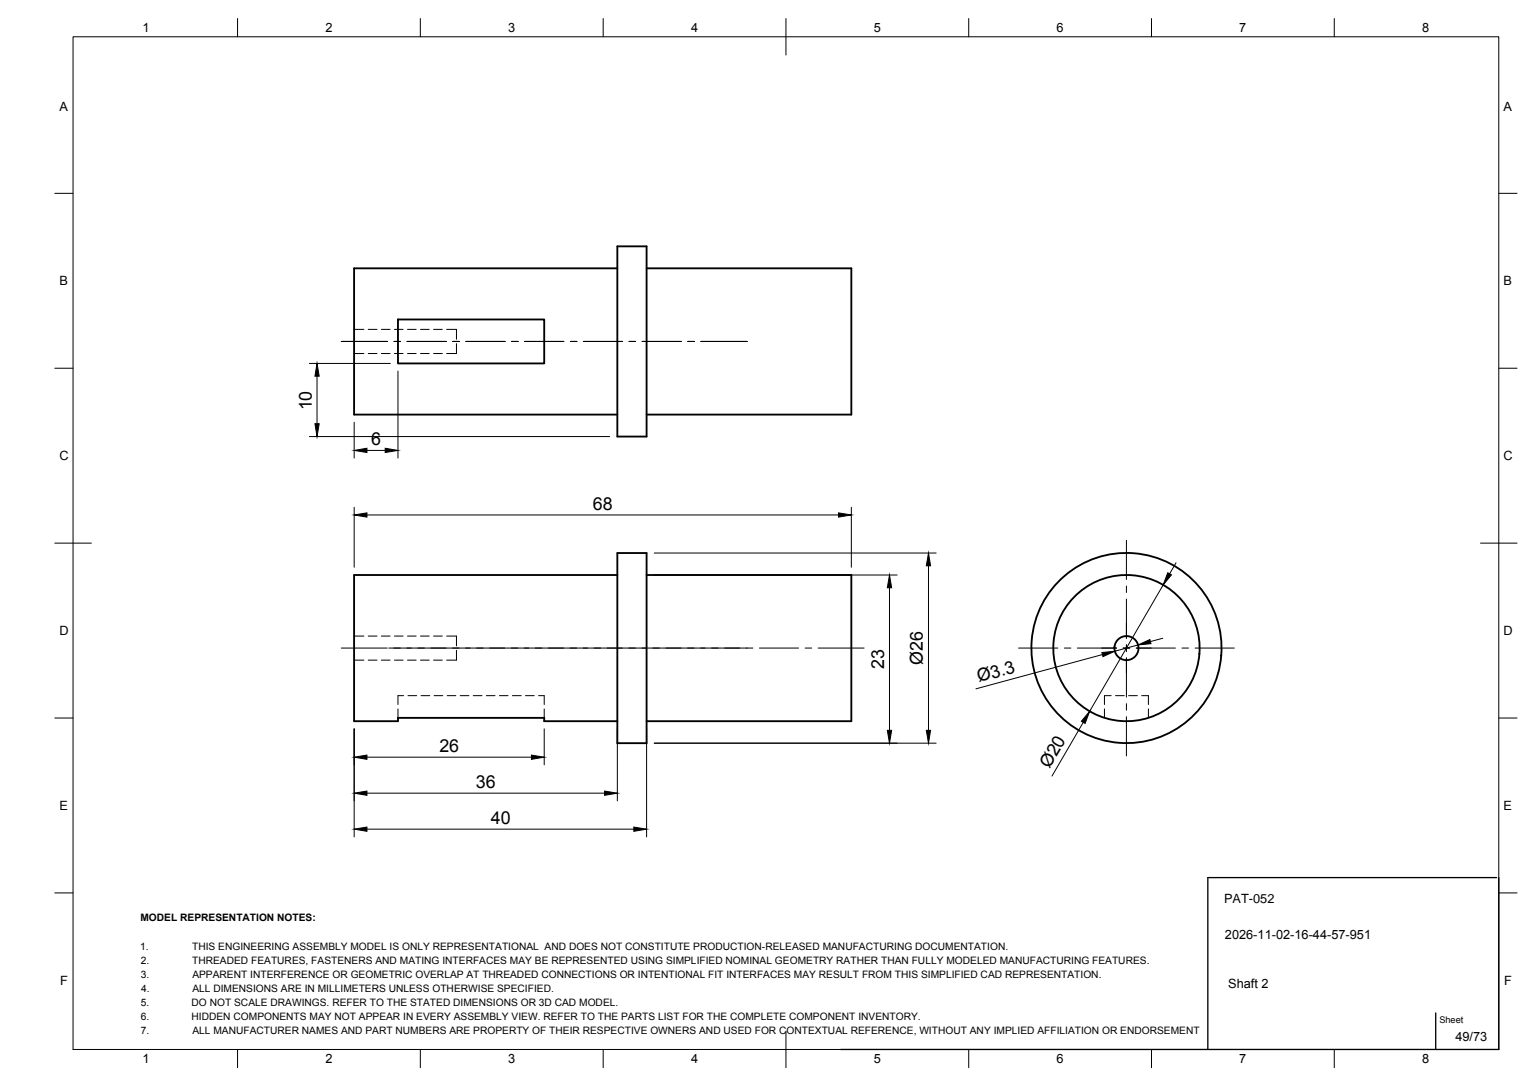
ISO-10303-21;
HEADER;
/* Generated by software containing ST-Developer
 * from STEP Tools, Inc. (www.steptools.com) 
 */

FILE_DESCRIPTION(
/* description */ ('Hand-crank gear train demonstrator'),
/* implementation_level */ '2;1');

FILE_NAME(
/* name */ 'Shaft 2.step',
/* time_stamp */ '2026-10-28T03:22:13-07:00',
/* author */ (''),
/* organization */ (''),
/* preprocessor_version */ 'ST-DEVELOPER v20.2',
/* originating_system */ 'Autodesk Translation Framework v15.17.0.0',
/* authorisation */ '');

FILE_SCHEMA (('AUTOMOTIVE_DESIGN { 1 0 10303 214 3 1 1 }'));
ENDSEC;

DATA;
#10=MECHANICAL_DESIGN_GEOMETRIC_PRESENTATION_REPRESENTATION('',(#1243),#62758);
#1100=SHAPE_REPRESENTATION_RELATIONSHIP('SRR','None',#63076,#1164);
#1164=ADVANCED_BREP_SHAPE_REPRESENTATION('',(#1318),#62730);
#1243=STYLED_ITEM('',(#63462),#1318);
#1318=MANIFOLD_SOLID_BREP('Body1',#16427);
#1572=FACE_BOUND('',#3806,.T.);
#1573=FACE_BOUND('',#3808,.T.);
#1574=FACE_BOUND('',#3812,.T.);
#1575=FACE_BOUND('',#3814,.T.);
#1937=PLANE('',#18140);
#1938=PLANE('',#18141);
#1939=PLANE('',#18142);
#1940=PLANE('',#18144);
#1941=PLANE('',#18145);
#1942=PLANE('',#18146);
#1943=PLANE('',#18148);
#1944=PLANE('',#18151);
#1945=PLANE('',#18159);
#1946=PLANE('',#18160);
#2632=FACE_OUTER_BOUND('',#3798,.T.);
#2633=FACE_OUTER_BOUND('',#3799,.T.);
#2634=FACE_OUTER_BOUND('',#3800,.T.);
#2635=FACE_OUTER_BOUND('',#3801,.T.);
#2636=FACE_OUTER_BOUND('',#3802,.T.);
#2637=FACE_OUTER_BOUND('',#3803,.T.);
#2638=FACE_OUTER_BOUND('',#3804,.T.);
#2639=FACE_OUTER_BOUND('',#3805,.T.);
#2640=FACE_OUTER_BOUND('',#3807,.T.);
#2641=FACE_OUTER_BOUND('',#3809,.T.);
#2642=FACE_OUTER_BOUND('',#3810,.T.);
#2643=FACE_OUTER_BOUND('',#3811,.T.);
#2644=FACE_OUTER_BOUND('',#3813,.T.);
#2645=FACE_OUTER_BOUND('',#3815,.T.);
#3798=EDGE_LOOP('',(#13023,#13024,#13025,#13026));
#3799=EDGE_LOOP('',(#13027));
#3800=EDGE_LOOP('',(#13028,#13029,#13030,#13031));
#3801=EDGE_LOOP('',(#13032,#13033,#13034,#13035));
#3802=EDGE_LOOP('',(#13036,#13037,#13038,#13039));
#3803=EDGE_LOOP('',(#13040,#13041,#13042,#13043));
#3804=EDGE_LOOP('',(#13044,#13045,#13046,#13047));
#3805=EDGE_LOOP('',(#13048));
#3806=EDGE_LOOP('',(#13049));
#3807=EDGE_LOOP('',(#13050));
#3808=EDGE_LOOP('',(#13051));
#3809=EDGE_LOOP('',(#13052,#13053,#13054,#13055));
#3810=EDGE_LOOP('',(#13056,#13057,#13058,#13059));
#3811=EDGE_LOOP('',(#13060,#13061,#13062,#13063));
#3812=EDGE_LOOP('',(#13064,#13065,#13066,#13067));
#3813=EDGE_LOOP('',(#13068));
#3814=EDGE_LOOP('',(#13069));
#3815=EDGE_LOOP('',(#13070));
#4930=LINE('',#26399,#6062);
#4931=LINE('',#26405,#6063);
#4932=LINE('',#26407,#6064);
#4933=LINE('',#26409,#6065);
#4934=LINE('',#26410,#6066);
#4935=LINE('',#26415,#6067);
#4936=LINE('',#26416,#6068);
#4937=LINE('',#26419,#6069);
#4938=LINE('',#26421,#6070);
#4939=LINE('',#26422,#6071);
#4940=LINE('',#26424,#6072);
#4941=LINE('',#26438,#6073);
#4942=LINE('',#26441,#6074);
#4943=LINE('',#26446,#6075);
#6062=VECTOR('',#21437,0.165);
#6063=VECTOR('',#21444,1.);
#6064=VECTOR('',#21445,1.);
#6065=VECTOR('',#21446,1.);
#6066=VECTOR('',#21447,1.);
#6067=VECTOR('',#21452,1.);
#6068=VECTOR('',#21453,1.);
#6069=VECTOR('',#21456,1.);
#6070=VECTOR('',#21457,1.);
#6071=VECTOR('',#21458,1.);
#6072=VECTOR('',#21461,1.);
#6073=VECTOR('',#21480,1.3);
#6074=VECTOR('',#21483,1.);
#6075=VECTOR('',#21490,1.);
#6964=CIRCLE('',#18138,0.165);
#6965=CIRCLE('',#18139,0.165);
#6966=CIRCLE('',#18143,1.);
#6967=CIRCLE('',#18147,1.);
#6968=CIRCLE('',#18149,1.3);
#6969=CIRCLE('',#18150,1.);
#6970=CIRCLE('',#18152,1.3);
#6971=CIRCLE('',#18153,1.);
#6972=CIRCLE('',#18156,1.);
#6973=CIRCLE('',#18158,1.);
#7955=VERTEX_POINT('',#26396);
#7956=VERTEX_POINT('',#26398);
#7957=VERTEX_POINT('',#26403);
#7958=VERTEX_POINT('',#26404);
#7959=VERTEX_POINT('',#26406);
#7960=VERTEX_POINT('',#26408);
#7961=VERTEX_POINT('',#26412);
#7962=VERTEX_POINT('',#26414);
#7963=VERTEX_POINT('',#26418);
#7964=VERTEX_POINT('',#26420);
#7965=VERTEX_POINT('',#26428);
#7966=VERTEX_POINT('',#26430);
#7967=VERTEX_POINT('',#26433);
#7968=VERTEX_POINT('',#26435);
#7969=VERTEX_POINT('',#26440);
#7970=VERTEX_POINT('',#26444);
#9763=EDGE_CURVE('',#7955,#7955,#6964,.T.);
#9764=EDGE_CURVE('',#7955,#7956,#4930,.T.);
#9765=EDGE_CURVE('',#7956,#7956,#6965,.T.);
#9766=EDGE_CURVE('',#7957,#7958,#4931,.T.);
#9767=EDGE_CURVE('',#7957,#7959,#4932,.T.);
#9768=EDGE_CURVE('',#7960,#7959,#4933,.T.);
#9769=EDGE_CURVE('',#7960,#7958,#4934,.T.);
#9770=EDGE_CURVE('',#7958,#7961,#6966,.T.);
#9771=EDGE_CURVE('',#7962,#7960,#4935,.T.);
#9772=EDGE_CURVE('',#7961,#7962,#4936,.T.);
#9773=EDGE_CURVE('',#7961,#7963,#4937,.T.);
#9774=EDGE_CURVE('',#7962,#7964,#4938,.T.);
#9775=EDGE_CURVE('',#7964,#7963,#4939,.T.);
#9776=EDGE_CURVE('',#7959,#7964,#4940,.T.);
#9777=EDGE_CURVE('',#7963,#7957,#6967,.T.);
#9778=EDGE_CURVE('',#7965,#7965,#6968,.T.);
#9779=EDGE_CURVE('',#7966,#7966,#6969,.T.);
#9780=EDGE_CURVE('',#7967,#7967,#6970,.T.);
#9781=EDGE_CURVE('',#7968,#7968,#6971,.T.);
#9782=EDGE_CURVE('',#7965,#7967,#4941,.T.);
#9783=EDGE_CURVE('',#7968,#7969,#4942,.T.);
#9784=EDGE_CURVE('',#7969,#7969,#6972,.T.);
#9785=EDGE_CURVE('',#7970,#7970,#6973,.T.);
#9786=EDGE_CURVE('',#7970,#7966,#4943,.T.);
#13023=ORIENTED_EDGE('',*,*,#9763,.F.);
#13024=ORIENTED_EDGE('',*,*,#9764,.T.);
#13025=ORIENTED_EDGE('',*,*,#9765,.F.);
#13026=ORIENTED_EDGE('',*,*,#9764,.F.);
#13027=ORIENTED_EDGE('',*,*,#9763,.T.);
#13028=ORIENTED_EDGE('',*,*,#9766,.F.);
#13029=ORIENTED_EDGE('',*,*,#9767,.T.);
#13030=ORIENTED_EDGE('',*,*,#9768,.F.);
#13031=ORIENTED_EDGE('',*,*,#9769,.T.);
#13032=ORIENTED_EDGE('',*,*,#9770,.F.);
#13033=ORIENTED_EDGE('',*,*,#9769,.F.);
#13034=ORIENTED_EDGE('',*,*,#9771,.F.);
#13035=ORIENTED_EDGE('',*,*,#9772,.F.);
#13036=ORIENTED_EDGE('',*,*,#9773,.F.);
#13037=ORIENTED_EDGE('',*,*,#9772,.T.);
#13038=ORIENTED_EDGE('',*,*,#9774,.T.);
#13039=ORIENTED_EDGE('',*,*,#9775,.T.);
#13040=ORIENTED_EDGE('',*,*,#9771,.T.);
#13041=ORIENTED_EDGE('',*,*,#9768,.T.);
#13042=ORIENTED_EDGE('',*,*,#9776,.T.);
#13043=ORIENTED_EDGE('',*,*,#9774,.F.);
#13044=ORIENTED_EDGE('',*,*,#9777,.F.);
#13045=ORIENTED_EDGE('',*,*,#9775,.F.);
#13046=ORIENTED_EDGE('',*,*,#9776,.F.);
#13047=ORIENTED_EDGE('',*,*,#9767,.F.);
#13048=ORIENTED_EDGE('',*,*,#9778,.T.);
#13049=ORIENTED_EDGE('',*,*,#9779,.F.);
#13050=ORIENTED_EDGE('',*,*,#9780,.F.);
#13051=ORIENTED_EDGE('',*,*,#9781,.F.);
#13052=ORIENTED_EDGE('',*,*,#9778,.F.);
#13053=ORIENTED_EDGE('',*,*,#9782,.T.);
#13054=ORIENTED_EDGE('',*,*,#9780,.T.);
#13055=ORIENTED_EDGE('',*,*,#9782,.F.);
#13056=ORIENTED_EDGE('',*,*,#9781,.T.);
#13057=ORIENTED_EDGE('',*,*,#9783,.T.);
#13058=ORIENTED_EDGE('',*,*,#9784,.T.);
#13059=ORIENTED_EDGE('',*,*,#9783,.F.);
#13060=ORIENTED_EDGE('',*,*,#9785,.F.);
#13061=ORIENTED_EDGE('',*,*,#9786,.T.);
#13062=ORIENTED_EDGE('',*,*,#9779,.T.);
#13063=ORIENTED_EDGE('',*,*,#9786,.F.);
#13064=ORIENTED_EDGE('',*,*,#9773,.T.);
#13065=ORIENTED_EDGE('',*,*,#9777,.T.);
#13066=ORIENTED_EDGE('',*,*,#9766,.T.);
#13067=ORIENTED_EDGE('',*,*,#9770,.T.);
#13068=ORIENTED_EDGE('',*,*,#9785,.T.);
#13069=ORIENTED_EDGE('',*,*,#9765,.T.);
#13070=ORIENTED_EDGE('',*,*,#9784,.F.);
#15318=CYLINDRICAL_SURFACE('',#18137,0.165);
#15319=CYLINDRICAL_SURFACE('',#18154,1.3);
#15320=CYLINDRICAL_SURFACE('',#18155,1.);
#15321=CYLINDRICAL_SURFACE('',#18157,1.);
#15942=ADVANCED_FACE('',(#2632),#15318,.F.);
#15943=ADVANCED_FACE('',(#2633),#1937,.T.);
#15944=ADVANCED_FACE('',(#2634),#1938,.F.);
#15945=ADVANCED_FACE('',(#2635),#1939,.T.);
#15946=ADVANCED_FACE('',(#2636),#1940,.F.);
#15947=ADVANCED_FACE('',(#2637),#1941,.F.);
#15948=ADVANCED_FACE('',(#2638),#1942,.F.);
#15949=ADVANCED_FACE('',(#2639,#1572),#1943,.T.);
#15950=ADVANCED_FACE('',(#2640,#1573),#1944,.F.);
#15951=ADVANCED_FACE('',(#2641),#15319,.T.);
#15952=ADVANCED_FACE('',(#2642),#15320,.T.);
#15953=ADVANCED_FACE('',(#2643,#1574),#15321,.T.);
#15954=ADVANCED_FACE('',(#2644,#1575),#1945,.T.);
#15955=ADVANCED_FACE('',(#2645),#1946,.F.);
#16427=CLOSED_SHELL('',(#15942,#15943,#15944,#15945,#15946,#15947,#15948,
#15949,#15950,#15951,#15952,#15953,#15954,#15955));
#18136=AXIS2_PLACEMENT_3D('',#26394,#21431,#21432);
#18137=AXIS2_PLACEMENT_3D('',#26395,#21433,#21434);
#18138=AXIS2_PLACEMENT_3D('',#26397,#21435,#21436);
#18139=AXIS2_PLACEMENT_3D('',#26400,#21438,#21439);
#18140=AXIS2_PLACEMENT_3D('',#26401,#21440,#21441);
#18141=AXIS2_PLACEMENT_3D('',#26402,#21442,#21443);
#18142=AXIS2_PLACEMENT_3D('',#26411,#21448,#21449);
#18143=AXIS2_PLACEMENT_3D('',#26413,#21450,#21451);
#18144=AXIS2_PLACEMENT_3D('',#26417,#21454,#21455);
#18145=AXIS2_PLACEMENT_3D('',#26423,#21459,#21460);
#18146=AXIS2_PLACEMENT_3D('',#26425,#21462,#21463);
#18147=AXIS2_PLACEMENT_3D('',#26426,#21464,#21465);
#18148=AXIS2_PLACEMENT_3D('',#26427,#21466,#21467);
#18149=AXIS2_PLACEMENT_3D('',#26429,#21468,#21469);
#18150=AXIS2_PLACEMENT_3D('',#26431,#21470,#21471);
#18151=AXIS2_PLACEMENT_3D('',#26432,#21472,#21473);
#18152=AXIS2_PLACEMENT_3D('',#26434,#21474,#21475);
#18153=AXIS2_PLACEMENT_3D('',#26436,#21476,#21477);
#18154=AXIS2_PLACEMENT_3D('',#26437,#21478,#21479);
#18155=AXIS2_PLACEMENT_3D('',#26439,#21481,#21482);
#18156=AXIS2_PLACEMENT_3D('',#26442,#21484,#21485);
#18157=AXIS2_PLACEMENT_3D('',#26443,#21486,#21487);
#18158=AXIS2_PLACEMENT_3D('',#26445,#21488,#21489);
#18159=AXIS2_PLACEMENT_3D('',#26447,#21491,#21492);
#18160=AXIS2_PLACEMENT_3D('',#26448,#21493,#21494);
#21431=DIRECTION('axis',(0.,0.,1.));
#21432=DIRECTION('refdir',(1.,0.,0.));
#21433=DIRECTION('center_axis',(0.,1.,0.));
#21434=DIRECTION('ref_axis',(1.,0.,0.));
#21435=DIRECTION('center_axis',(0.,1.,0.));
#21436=DIRECTION('ref_axis',(1.,0.,0.));
#21437=DIRECTION('',(0.,1.,0.));
#21438=DIRECTION('center_axis',(0.,-1.,0.));
#21439=DIRECTION('ref_axis',(1.,0.,0.));
#21440=DIRECTION('center_axis',(0.,1.,0.));
#21441=DIRECTION('ref_axis',(1.,0.,0.));
#21442=DIRECTION('center_axis',(-1.,0.,0.));
#21443=DIRECTION('ref_axis',(0.,0.,1.));
#21444=DIRECTION('',(0.,-1.,0.));
#21445=DIRECTION('',(0.,0.,1.));
#21446=DIRECTION('',(0.,1.,0.));
#21447=DIRECTION('',(0.,0.,-1.));
#21448=DIRECTION('center_axis',(0.,1.,0.));
#21449=DIRECTION('ref_axis',(1.,0.,0.));
#21450=DIRECTION('center_axis',(0.,-1.,0.));
#21451=DIRECTION('ref_axis',(1.,0.,0.));
#21452=DIRECTION('',(-1.,0.,0.));
#21453=DIRECTION('',(0.,0.,1.));
#21454=DIRECTION('center_axis',(1.,0.,0.));
#21455=DIRECTION('ref_axis',(0.,0.,-1.));
#21456=DIRECTION('',(0.,1.,0.));
#21457=DIRECTION('',(0.,1.,0.));
#21458=DIRECTION('',(0.,0.,-1.));
#21459=DIRECTION('center_axis',(0.,0.,1.));
#21460=DIRECTION('ref_axis',(1.,0.,0.));
#21461=DIRECTION('',(1.,0.,0.));
#21462=DIRECTION('center_axis',(0.,1.,0.));
#21463=DIRECTION('ref_axis',(0.,0.,1.));
#21464=DIRECTION('center_axis',(0.,1.,0.));
#21465=DIRECTION('ref_axis',(1.,0.,0.));
#21466=DIRECTION('center_axis',(0.,1.,0.));
#21467=DIRECTION('ref_axis',(1.,0.,0.));
#21468=DIRECTION('center_axis',(0.,1.,0.));
#21469=DIRECTION('ref_axis',(1.,0.,0.));
#21470=DIRECTION('center_axis',(0.,1.,0.));
#21471=DIRECTION('ref_axis',(1.,0.,0.));
#21472=DIRECTION('center_axis',(0.,1.,0.));
#21473=DIRECTION('ref_axis',(1.,0.,0.));
#21474=DIRECTION('center_axis',(0.,1.,0.));
#21475=DIRECTION('ref_axis',(1.,0.,0.));
#21476=DIRECTION('center_axis',(0.,-1.,0.));
#21477=DIRECTION('ref_axis',(1.,0.,0.));
#21478=DIRECTION('center_axis',(0.,1.,0.));
#21479=DIRECTION('ref_axis',(1.,0.,0.));
#21480=DIRECTION('',(0.,-1.,0.));
#21481=DIRECTION('center_axis',(0.,1.,0.));
#21482=DIRECTION('ref_axis',(1.,0.,0.));
#21483=DIRECTION('',(0.,-1.,0.));
#21484=DIRECTION('center_axis',(0.,1.,0.));
#21485=DIRECTION('ref_axis',(1.,0.,0.));
#21486=DIRECTION('center_axis',(0.,1.,0.));
#21487=DIRECTION('ref_axis',(1.,0.,0.));
#21488=DIRECTION('center_axis',(0.,1.,0.));
#21489=DIRECTION('ref_axis',(1.,0.,0.));
#21490=DIRECTION('',(0.,-1.,0.));
#21491=DIRECTION('center_axis',(0.,1.,0.));
#21492=DIRECTION('ref_axis',(1.,0.,0.));
#21493=DIRECTION('center_axis',(0.,1.,0.));
#21494=DIRECTION('ref_axis',(1.,0.,0.));
#26394=CARTESIAN_POINT('',(0.,0.,0.));
#26395=CARTESIAN_POINT('Origin',(6.,1.8,9.));
#26396=CARTESIAN_POINT('',(5.835,1.8,9.));
#26397=CARTESIAN_POINT('Origin',(6.,1.8,9.));
#26398=CARTESIAN_POINT('',(5.835,3.2,9.));
#26399=CARTESIAN_POINT('',(5.835,1.8,9.));
#26400=CARTESIAN_POINT('Origin',(6.,3.2,9.));
#26401=CARTESIAN_POINT('Origin',(6.,1.8,9.));
#26402=CARTESIAN_POINT('Origin',(5.7,0.6,7.));
#26403=CARTESIAN_POINT('',(5.7,2.6,8.04606079858305));
#26404=CARTESIAN_POINT('',(5.7,0.6,8.04606079858305));
#26405=CARTESIAN_POINT('',(5.7,-3.6,8.04606079858305));
#26406=CARTESIAN_POINT('',(5.7,2.6,8.35));
#26407=CARTESIAN_POINT('',(5.7,2.6,8.35));
#26408=CARTESIAN_POINT('',(5.7,0.6,8.35));
#26409=CARTESIAN_POINT('',(5.7,0.6,8.35));
#26410=CARTESIAN_POINT('',(5.7,0.6,8.35));
#26411=CARTESIAN_POINT('Origin',(6.,0.6,7.675));
#26412=CARTESIAN_POINT('',(6.3,0.6,8.04606079858305));
#26413=CARTESIAN_POINT('Origin',(6.,0.6,9.));
#26414=CARTESIAN_POINT('',(6.3,0.6,8.35));
#26415=CARTESIAN_POINT('',(6.3,0.6,8.35));
#26416=CARTESIAN_POINT('',(6.3,0.6,7.));
#26417=CARTESIAN_POINT('Origin',(6.3,0.6,8.35));
#26418=CARTESIAN_POINT('',(6.3,2.6,8.04606079858305));
#26419=CARTESIAN_POINT('',(6.3,-3.6,8.04606079858305));
#26420=CARTESIAN_POINT('',(6.3,2.6,8.35));
#26421=CARTESIAN_POINT('',(6.3,0.6,8.35));
#26422=CARTESIAN_POINT('',(6.3,2.6,7.));
#26423=CARTESIAN_POINT('Origin',(5.7,0.6,8.35));
#26424=CARTESIAN_POINT('',(6.3,2.6,8.35));
#26425=CARTESIAN_POINT('Origin',(6.,2.6,7.675));
#26426=CARTESIAN_POINT('Origin',(6.,2.6,9.));
#26427=CARTESIAN_POINT('Origin',(6.,-0.4,9.));
#26428=CARTESIAN_POINT('',(4.7,-0.4,9.));
#26429=CARTESIAN_POINT('Origin',(6.,-0.4,9.));
#26430=CARTESIAN_POINT('',(5.,-0.4,9.));
#26431=CARTESIAN_POINT('Origin',(6.,-0.4,9.));
#26432=CARTESIAN_POINT('Origin',(6.,-0.8,9.));
#26433=CARTESIAN_POINT('',(4.7,-0.8,9.));
#26434=CARTESIAN_POINT('Origin',(6.,-0.8,9.));
#26435=CARTESIAN_POINT('',(5.,-0.8,9.));
#26436=CARTESIAN_POINT('Origin',(6.,-0.8,9.));
#26437=CARTESIAN_POINT('Origin',(6.,-0.8,9.));
#26438=CARTESIAN_POINT('',(4.7,-0.8,9.));
#26439=CARTESIAN_POINT('Origin',(6.,-3.6,9.));
#26440=CARTESIAN_POINT('',(5.,-3.6,9.));
#26441=CARTESIAN_POINT('',(5.,-3.6,9.));
#26442=CARTESIAN_POINT('Origin',(6.,-3.6,9.));
#26443=CARTESIAN_POINT('Origin',(6.,-3.6,9.));
#26444=CARTESIAN_POINT('',(5.,3.2,9.));
#26445=CARTESIAN_POINT('Origin',(6.,3.2,9.));
#26446=CARTESIAN_POINT('',(5.,-3.6,9.));
#26447=CARTESIAN_POINT('Origin',(6.,3.2,9.));
#26448=CARTESIAN_POINT('Origin',(6.,-3.6,9.));
#62656=UNCERTAINTY_MEASURE_WITH_UNIT(LENGTH_MEASURE(0.001),#62759,
'DISTANCE_ACCURACY_VALUE',
'Maximum model space distance between geometric entities at asserted c
onnectivities');
#62684=UNCERTAINTY_MEASURE_WITH_UNIT(LENGTH_MEASURE(0.001),#62759,
'DISTANCE_ACCURACY_VALUE',
'Maximum model space distance between geometric entities at asserted c
onnectivities');
#62730=(
GEOMETRIC_REPRESENTATION_CONTEXT(3)
GLOBAL_UNCERTAINTY_ASSIGNED_CONTEXT((#62656))
GLOBAL_UNIT_ASSIGNED_CONTEXT((#62759,#62761,#62762))
REPRESENTATION_CONTEXT('','3D')
);
#62758=(
GEOMETRIC_REPRESENTATION_CONTEXT(3)
GLOBAL_UNCERTAINTY_ASSIGNED_CONTEXT((#62684))
GLOBAL_UNIT_ASSIGNED_CONTEXT((#62759,#62761,#62762))
REPRESENTATION_CONTEXT('','3D')
);
#62759=(
LENGTH_UNIT()
NAMED_UNIT(*)
SI_UNIT(.CENTI.,.METRE.)
);
#62761=(
NAMED_UNIT(*)
PLANE_ANGLE_UNIT()
SI_UNIT($,.RADIAN.)
);
#62762=(
NAMED_UNIT(*)
SI_UNIT($,.STERADIAN.)
SOLID_ANGLE_UNIT()
);
#62808=SHAPE_DEFINITION_REPRESENTATION(#62891,#63076);
#62891=PRODUCT_DEFINITION_SHAPE('',$,#63150);
#63076=SHAPE_REPRESENTATION('',(#18136),#62730);
#63104=PRODUCT_DEFINITION_CONTEXT('part definition',#63325,'design');
#63150=PRODUCT_DEFINITION('Shaft 2','Shaft 2',#63223,#63104);
#63223=PRODUCT_DEFINITION_FORMATION('',$,#63372);
#63325=APPLICATION_CONTEXT(
'Core Data for Automotive Mechanical Design Process');
#63326=PRODUCT_CONTEXT('part definition',#63325,'mechanical');
#63372=PRODUCT('Shaft 2','Shaft 2','Shaft 2',(#63326));
#63456=COLOUR_RGB('Grey',0.48,0.52,0.57);
#63457=FILL_AREA_STYLE_COLOUR('',#63456);
#63458=FILL_AREA_STYLE('',(#63457));
#63459=SURFACE_STYLE_FILL_AREA(#63458);
#63460=SURFACE_SIDE_STYLE('',(#63459));
#63461=SURFACE_STYLE_USAGE(.BOTH.,#63460);
#63462=PRESENTATION_STYLE_ASSIGNMENT((#63461));
ENDSEC;
END-ISO-10303-21;
